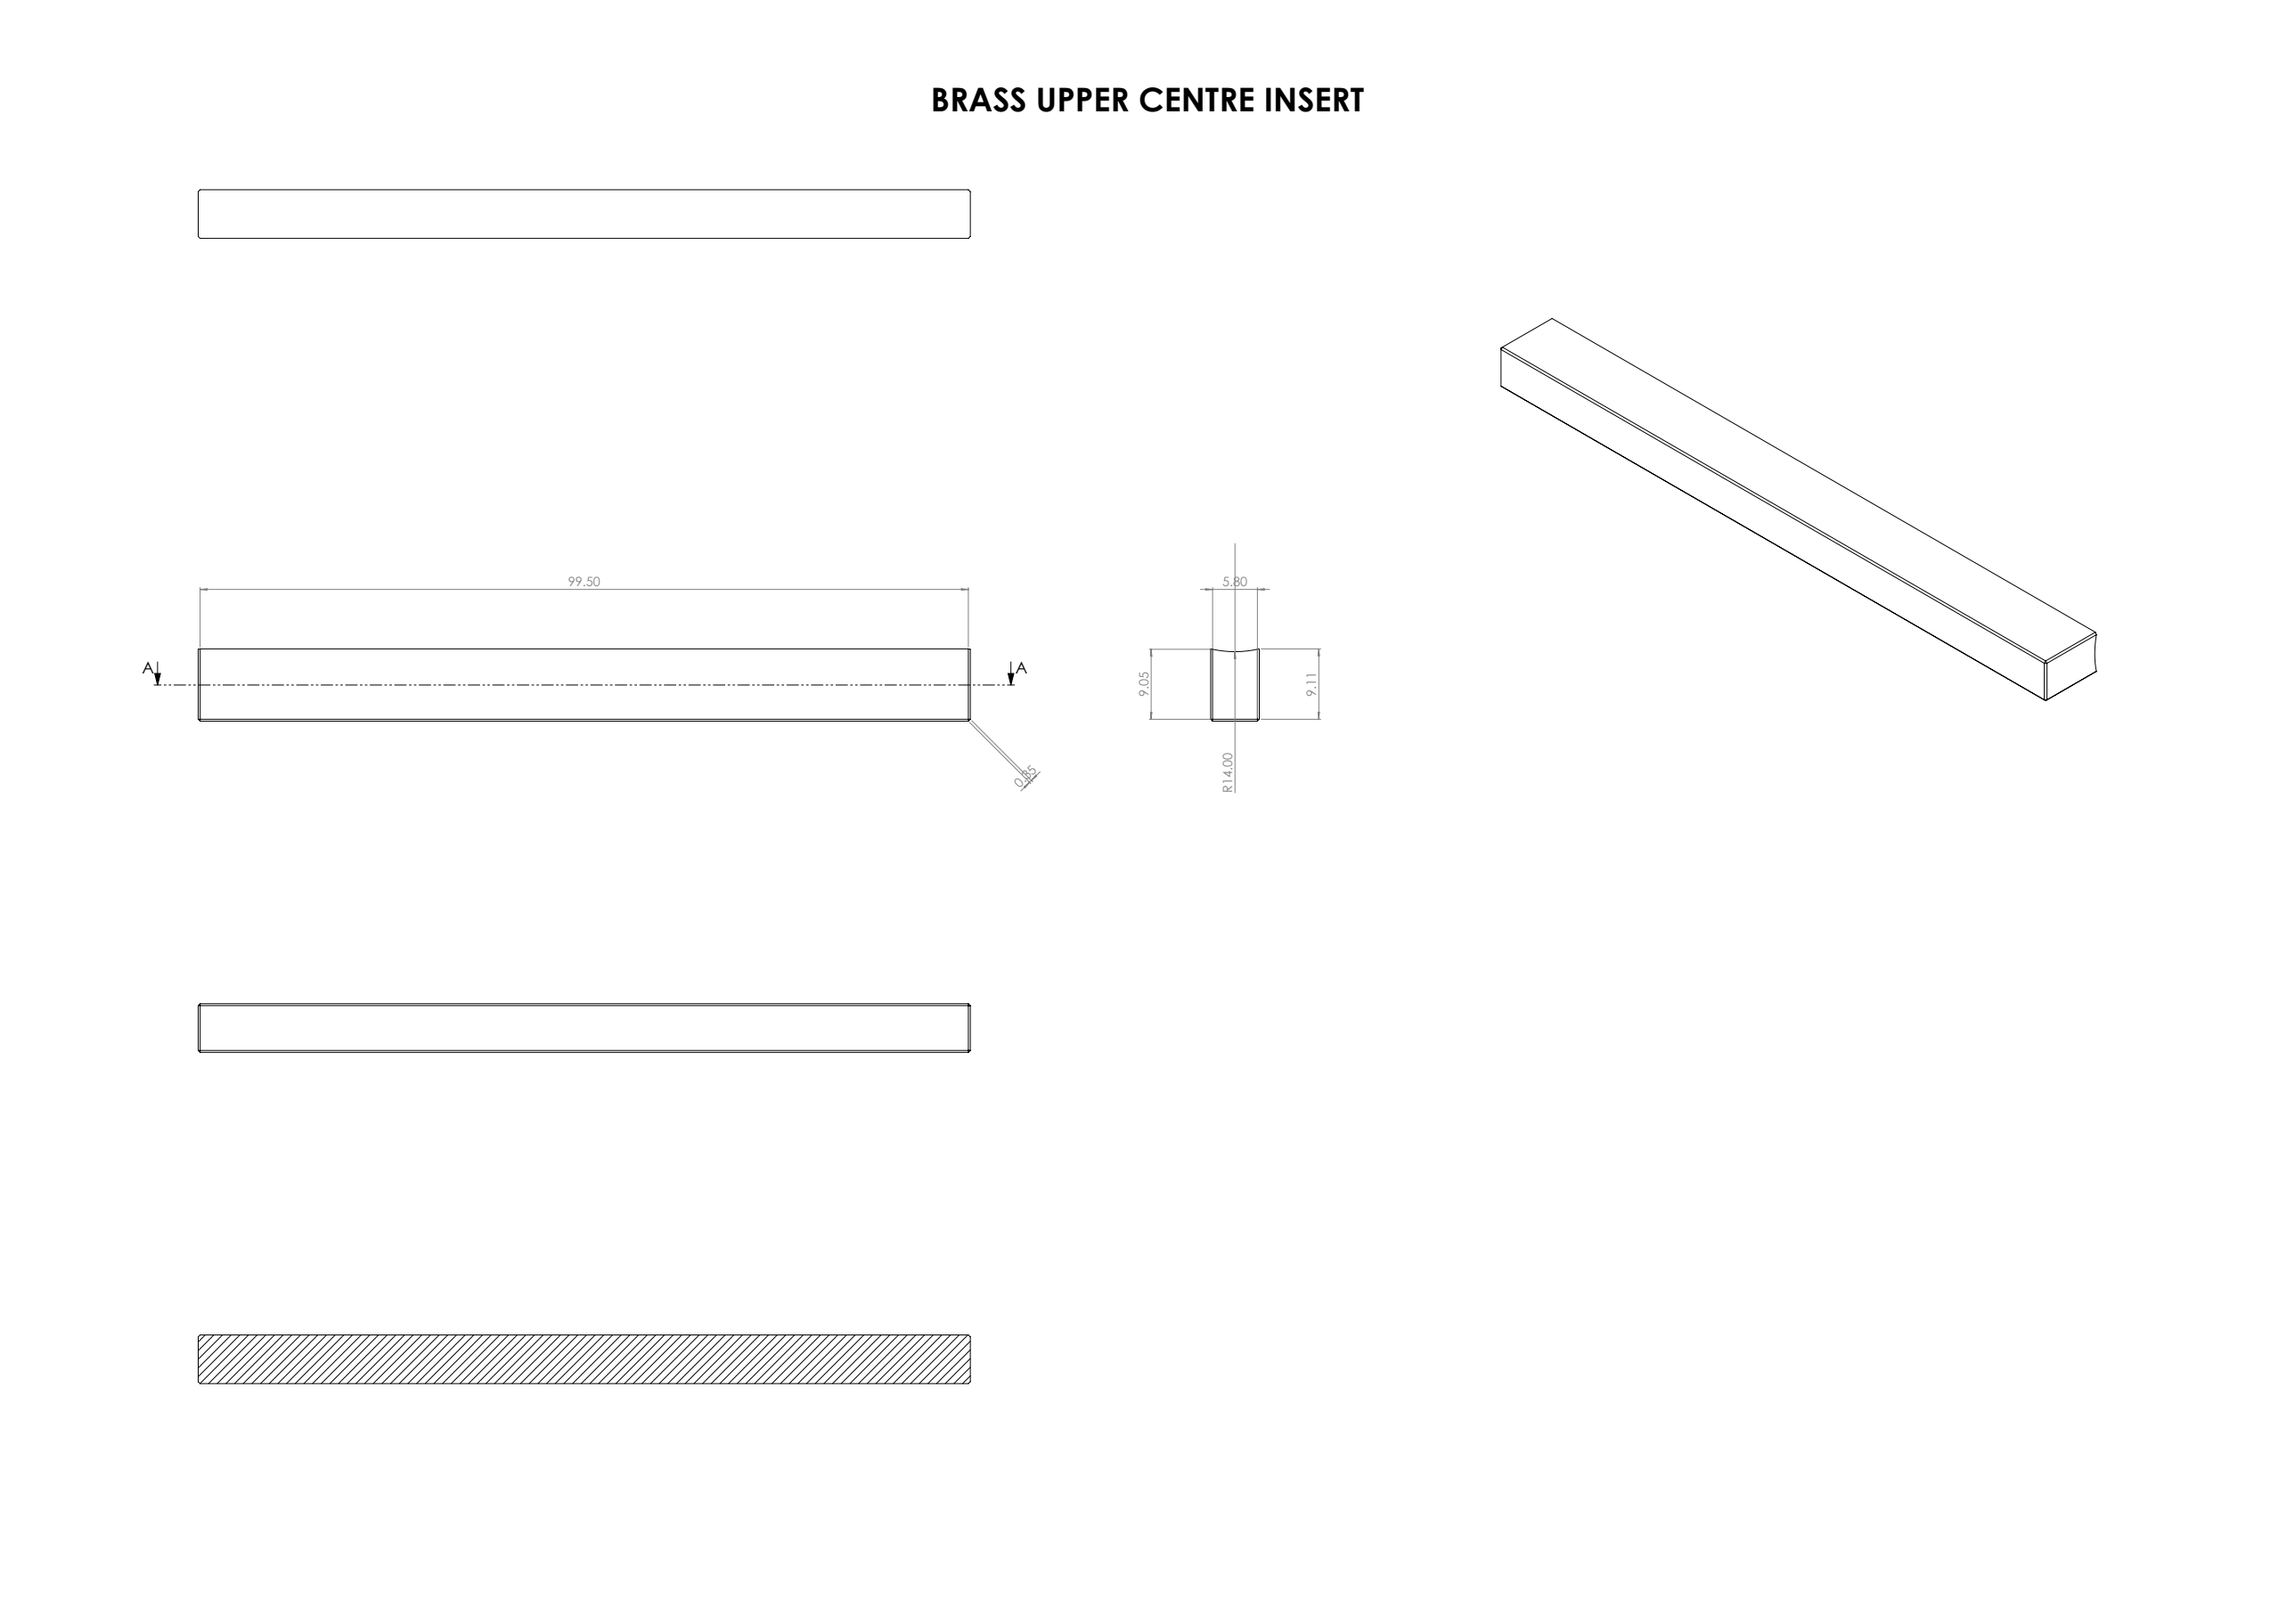
ISO-10303-21;
HEADER;
/* Generated by software containing ST-Developer
 * from STEP Tools, Inc. (www.steptools.com) 
 */

FILE_DESCRIPTION(
/* description */ (''),
/* implementation_level */ '2;1');

FILE_NAME(
/* name */ '13_Brass_Upper_Centre_Insert.step',
/* time_stamp */ '2026-10-21T01:59:45-07:00',
/* author */ (''),
/* organization */ (''),
/* preprocessor_version */ 'ST-DEVELOPER v20.2',
/* originating_system */ 'Autodesk Translation Framework v15.15.0.0',
/* authorisation */ '');

FILE_SCHEMA (('AUTOMOTIVE_DESIGN { 1 0 10303 214 3 1 1 }'));
ENDSEC;

DATA;
#10=MECHANICAL_DESIGN_GEOMETRIC_PRESENTATION_REPRESENTATION('',(#464),#18281);
#438=SHAPE_REPRESENTATION_RELATIONSHIP('SRR','None',#18340,#451);
#451=ADVANCED_BREP_SHAPE_REPRESENTATION('',(#482),#18269);
#464=STYLED_ITEM('',(#18467),#482);
#482=MANIFOLD_SOLID_BREP('Body1',#9086);
#498=CYLINDRICAL_SURFACE('',#9298,14.);
#637=CIRCLE('',#9296,14.);
#638=CIRCLE('',#9299,14.);
#826=ELLIPSE('',#9281,19.7989898732233,14.);
#827=ELLIPSE('',#9286,19.7989898732233,14.);
#828=ELLIPSE('',#9291,19.7989898732235,14.);
#829=ELLIPSE('',#9293,19.7989898732235,14.);
#863=FACE_OUTER_BOUND('',#1391,.T.);
#864=FACE_OUTER_BOUND('',#1392,.T.);
#865=FACE_OUTER_BOUND('',#1393,.T.);
#866=FACE_OUTER_BOUND('',#1394,.T.);
#867=FACE_OUTER_BOUND('',#1395,.T.);
#868=FACE_OUTER_BOUND('',#1396,.T.);
#869=FACE_OUTER_BOUND('',#1397,.T.);
#870=FACE_OUTER_BOUND('',#1398,.T.);
#871=FACE_OUTER_BOUND('',#1399,.T.);
#872=FACE_OUTER_BOUND('',#1400,.T.);
#873=FACE_OUTER_BOUND('',#1401,.T.);
#874=FACE_OUTER_BOUND('',#1402,.T.);
#875=FACE_OUTER_BOUND('',#1403,.T.);
#876=FACE_OUTER_BOUND('',#1404,.T.);
#877=FACE_OUTER_BOUND('',#1405,.T.);
#878=FACE_OUTER_BOUND('',#1406,.T.);
#879=FACE_OUTER_BOUND('',#1407,.T.);
#880=FACE_OUTER_BOUND('',#1408,.T.);
#1391=EDGE_LOOP('',(#5782,#5783,#5784));
#1392=EDGE_LOOP('',(#5785,#5786,#5787));
#1393=EDGE_LOOP('',(#5788,#5789,#5790,#5791));
#1394=EDGE_LOOP('',(#5792,#5793,#5794,#5795));
#1395=EDGE_LOOP('',(#5796,#5797,#5798));
#1396=EDGE_LOOP('',(#5799,#5800,#5801));
#1397=EDGE_LOOP('',(#5802,#5803,#5804,#5805));
#1398=EDGE_LOOP('',(#5806,#5807,#5808,#5809));
#1399=EDGE_LOOP('',(#5810,#5811,#5812,#5813));
#1400=EDGE_LOOP('',(#5814,#5815,#5816,#5817));
#1401=EDGE_LOOP('',(#5818,#5819,#5820,#5821));
#1402=EDGE_LOOP('',(#5822,#5823,#5824,#5825));
#1403=EDGE_LOOP('',(#5826,#5827,#5828,#5829));
#1404=EDGE_LOOP('',(#5830,#5831,#5832,#5833));
#1405=EDGE_LOOP('',(#5834,#5835,#5836,#5837));
#1406=EDGE_LOOP('',(#5838,#5839,#5840,#5841,#5842,#5843,#5844,#5845));
#1407=EDGE_LOOP('',(#5846,#5847,#5848,#5849));
#1408=EDGE_LOOP('',(#5850,#5851,#5852,#5853));
#1969=LINE('',#12369,#2814);
#1970=LINE('',#12371,#2815);
#1971=LINE('',#12372,#2816);
#1972=LINE('',#12376,#2817);
#1973=LINE('',#12378,#2818);
#1974=LINE('',#12379,#2819);
#1975=LINE('',#12384,#2820);
#1976=LINE('',#12385,#2821);
#1977=LINE('',#12387,#2822);
#1978=LINE('',#12388,#2823);
#1979=LINE('',#12392,#2824);
#1980=LINE('',#12394,#2825);
#1981=LINE('',#12395,#2826);
#1982=LINE('',#12399,#2827);
#1983=LINE('',#12401,#2828);
#1984=LINE('',#12402,#2829);
#1985=LINE('',#12407,#2830);
#1986=LINE('',#12408,#2831);
#1987=LINE('',#12410,#2832);
#1988=LINE('',#12411,#2833);
#1989=LINE('',#12413,#2834);
#1990=LINE('',#12414,#2835);
#1991=LINE('',#12416,#2836);
#1992=LINE('',#12417,#2837);
#1993=LINE('',#12422,#2838);
#1994=LINE('',#12423,#2839);
#1995=LINE('',#12428,#2840);
#1996=LINE('',#12429,#2841);
#1997=LINE('',#12431,#2842);
#1998=LINE('',#12436,#2843);
#2814=VECTOR('',#10077,10.);
#2815=VECTOR('',#10078,10.);
#2816=VECTOR('',#10079,10.);
#2817=VECTOR('',#10082,10.);
#2818=VECTOR('',#10083,10.);
#2819=VECTOR('',#10084,10.);
#2820=VECTOR('',#10089,10.);
#2821=VECTOR('',#10090,10.);
#2822=VECTOR('',#10093,10.);
#2823=VECTOR('',#10094,10.);
#2824=VECTOR('',#10097,10.);
#2825=VECTOR('',#10098,10.);
#2826=VECTOR('',#10099,10.);
#2827=VECTOR('',#10102,10.);
#2828=VECTOR('',#10103,10.);
#2829=VECTOR('',#10104,10.);
#2830=VECTOR('',#10109,10.);
#2831=VECTOR('',#10110,10.);
#2832=VECTOR('',#10113,10.);
#2833=VECTOR('',#10114,10.);
#2834=VECTOR('',#10117,10.);
#2835=VECTOR('',#10118,10.);
#2836=VECTOR('',#10121,10.);
#2837=VECTOR('',#10122,10.);
#2838=VECTOR('',#10127,10.);
#2839=VECTOR('',#10128,10.);
#2840=VECTOR('',#10133,10.);
#2841=VECTOR('',#10134,10.);
#2842=VECTOR('',#10137,10.);
#2843=VECTOR('',#10146,10.);
#3652=VERTEX_POINT('',#12367);
#3653=VERTEX_POINT('',#12368);
#3654=VERTEX_POINT('',#12370);
#3655=VERTEX_POINT('',#12374);
#3656=VERTEX_POINT('',#12375);
#3657=VERTEX_POINT('',#12377);
#3658=VERTEX_POINT('',#12381);
#3659=VERTEX_POINT('',#12382);
#3660=VERTEX_POINT('',#12390);
#3661=VERTEX_POINT('',#12391);
#3662=VERTEX_POINT('',#12393);
#3663=VERTEX_POINT('',#12397);
#3664=VERTEX_POINT('',#12398);
#3665=VERTEX_POINT('',#12400);
#3666=VERTEX_POINT('',#12404);
#3667=VERTEX_POINT('',#12405);
#3668=VERTEX_POINT('',#12419);
#3669=VERTEX_POINT('',#12420);
#3670=VERTEX_POINT('',#12425);
#3671=VERTEX_POINT('',#12426);
#4463=EDGE_CURVE('',#3652,#3653,#1969,.T.);
#4464=EDGE_CURVE('',#3654,#3652,#1970,.T.);
#4465=EDGE_CURVE('',#3653,#3654,#1971,.T.);
#4466=EDGE_CURVE('',#3655,#3656,#1972,.T.);
#4467=EDGE_CURVE('',#3657,#3655,#1973,.T.);
#4468=EDGE_CURVE('',#3656,#3657,#1974,.T.);
#4469=EDGE_CURVE('',#3658,#3659,#826,.T.);
#4470=EDGE_CURVE('',#3659,#3657,#1975,.T.);
#4471=EDGE_CURVE('',#3655,#3658,#1976,.T.);
#4472=EDGE_CURVE('',#3652,#3656,#1977,.T.);
#4473=EDGE_CURVE('',#3657,#3654,#1978,.T.);
#4474=EDGE_CURVE('',#3660,#3661,#1979,.T.);
#4475=EDGE_CURVE('',#3662,#3660,#1980,.T.);
#4476=EDGE_CURVE('',#3661,#3662,#1981,.T.);
#4477=EDGE_CURVE('',#3663,#3664,#1982,.T.);
#4478=EDGE_CURVE('',#3665,#3663,#1983,.T.);
#4479=EDGE_CURVE('',#3664,#3665,#1984,.T.);
#4480=EDGE_CURVE('',#3666,#3667,#827,.T.);
#4481=EDGE_CURVE('',#3667,#3665,#1985,.T.);
#4482=EDGE_CURVE('',#3663,#3666,#1986,.T.);
#4483=EDGE_CURVE('',#3656,#3664,#1987,.T.);
#4484=EDGE_CURVE('',#3665,#3655,#1988,.T.);
#4485=EDGE_CURVE('',#3660,#3663,#1989,.T.);
#4486=EDGE_CURVE('',#3664,#3662,#1990,.T.);
#4487=EDGE_CURVE('',#3653,#3661,#1991,.T.);
#4488=EDGE_CURVE('',#3662,#3652,#1992,.T.);
#4489=EDGE_CURVE('',#3668,#3669,#828,.T.);
#4490=EDGE_CURVE('',#3669,#3660,#1993,.T.);
#4491=EDGE_CURVE('',#3661,#3668,#1994,.T.);
#4492=EDGE_CURVE('',#3670,#3671,#829,.T.);
#4493=EDGE_CURVE('',#3671,#3653,#1995,.T.);
#4494=EDGE_CURVE('',#3654,#3670,#1996,.T.);
#4495=EDGE_CURVE('',#3669,#3666,#1997,.T.);
#4496=EDGE_CURVE('',#3671,#3668,#637,.T.);
#4497=EDGE_CURVE('',#3659,#3670,#1998,.T.);
#4498=EDGE_CURVE('',#3667,#3658,#638,.T.);
#5782=ORIENTED_EDGE('',*,*,#4463,.F.);
#5783=ORIENTED_EDGE('',*,*,#4464,.F.);
#5784=ORIENTED_EDGE('',*,*,#4465,.F.);
#5785=ORIENTED_EDGE('',*,*,#4466,.F.);
#5786=ORIENTED_EDGE('',*,*,#4467,.F.);
#5787=ORIENTED_EDGE('',*,*,#4468,.F.);
#5788=ORIENTED_EDGE('',*,*,#4469,.T.);
#5789=ORIENTED_EDGE('',*,*,#4470,.T.);
#5790=ORIENTED_EDGE('',*,*,#4467,.T.);
#5791=ORIENTED_EDGE('',*,*,#4471,.T.);
#5792=ORIENTED_EDGE('',*,*,#4464,.T.);
#5793=ORIENTED_EDGE('',*,*,#4472,.T.);
#5794=ORIENTED_EDGE('',*,*,#4468,.T.);
#5795=ORIENTED_EDGE('',*,*,#4473,.T.);
#5796=ORIENTED_EDGE('',*,*,#4474,.F.);
#5797=ORIENTED_EDGE('',*,*,#4475,.F.);
#5798=ORIENTED_EDGE('',*,*,#4476,.F.);
#5799=ORIENTED_EDGE('',*,*,#4477,.F.);
#5800=ORIENTED_EDGE('',*,*,#4478,.F.);
#5801=ORIENTED_EDGE('',*,*,#4479,.F.);
#5802=ORIENTED_EDGE('',*,*,#4480,.T.);
#5803=ORIENTED_EDGE('',*,*,#4481,.T.);
#5804=ORIENTED_EDGE('',*,*,#4478,.T.);
#5805=ORIENTED_EDGE('',*,*,#4482,.T.);
#5806=ORIENTED_EDGE('',*,*,#4466,.T.);
#5807=ORIENTED_EDGE('',*,*,#4483,.T.);
#5808=ORIENTED_EDGE('',*,*,#4479,.T.);
#5809=ORIENTED_EDGE('',*,*,#4484,.T.);
#5810=ORIENTED_EDGE('',*,*,#4475,.T.);
#5811=ORIENTED_EDGE('',*,*,#4485,.T.);
#5812=ORIENTED_EDGE('',*,*,#4477,.T.);
#5813=ORIENTED_EDGE('',*,*,#4486,.T.);
#5814=ORIENTED_EDGE('',*,*,#4463,.T.);
#5815=ORIENTED_EDGE('',*,*,#4487,.T.);
#5816=ORIENTED_EDGE('',*,*,#4476,.T.);
#5817=ORIENTED_EDGE('',*,*,#4488,.T.);
#5818=ORIENTED_EDGE('',*,*,#4489,.T.);
#5819=ORIENTED_EDGE('',*,*,#4490,.T.);
#5820=ORIENTED_EDGE('',*,*,#4474,.T.);
#5821=ORIENTED_EDGE('',*,*,#4491,.T.);
#5822=ORIENTED_EDGE('',*,*,#4492,.T.);
#5823=ORIENTED_EDGE('',*,*,#4493,.T.);
#5824=ORIENTED_EDGE('',*,*,#4465,.T.);
#5825=ORIENTED_EDGE('',*,*,#4494,.T.);
#5826=ORIENTED_EDGE('',*,*,#4482,.F.);
#5827=ORIENTED_EDGE('',*,*,#4485,.F.);
#5828=ORIENTED_EDGE('',*,*,#4490,.F.);
#5829=ORIENTED_EDGE('',*,*,#4495,.T.);
#5830=ORIENTED_EDGE('',*,*,#4491,.F.);
#5831=ORIENTED_EDGE('',*,*,#4487,.F.);
#5832=ORIENTED_EDGE('',*,*,#4493,.F.);
#5833=ORIENTED_EDGE('',*,*,#4496,.T.);
#5834=ORIENTED_EDGE('',*,*,#4472,.F.);
#5835=ORIENTED_EDGE('',*,*,#4488,.F.);
#5836=ORIENTED_EDGE('',*,*,#4486,.F.);
#5837=ORIENTED_EDGE('',*,*,#4483,.F.);
#5838=ORIENTED_EDGE('',*,*,#4480,.F.);
#5839=ORIENTED_EDGE('',*,*,#4495,.F.);
#5840=ORIENTED_EDGE('',*,*,#4489,.F.);
#5841=ORIENTED_EDGE('',*,*,#4496,.F.);
#5842=ORIENTED_EDGE('',*,*,#4492,.F.);
#5843=ORIENTED_EDGE('',*,*,#4497,.F.);
#5844=ORIENTED_EDGE('',*,*,#4469,.F.);
#5845=ORIENTED_EDGE('',*,*,#4498,.F.);
#5846=ORIENTED_EDGE('',*,*,#4481,.F.);
#5847=ORIENTED_EDGE('',*,*,#4498,.T.);
#5848=ORIENTED_EDGE('',*,*,#4471,.F.);
#5849=ORIENTED_EDGE('',*,*,#4484,.F.);
#5850=ORIENTED_EDGE('',*,*,#4470,.F.);
#5851=ORIENTED_EDGE('',*,*,#4497,.T.);
#5852=ORIENTED_EDGE('',*,*,#4494,.F.);
#5853=ORIENTED_EDGE('',*,*,#4473,.F.);
#8257=PLANE('',#9278);
#8258=PLANE('',#9279);
#8259=PLANE('',#9280);
#8260=PLANE('',#9282);
#8261=PLANE('',#9283);
#8262=PLANE('',#9284);
#8263=PLANE('',#9285);
#8264=PLANE('',#9287);
#8265=PLANE('',#9288);
#8266=PLANE('',#9289);
#8267=PLANE('',#9290);
#8268=PLANE('',#9292);
#8269=PLANE('',#9294);
#8270=PLANE('',#9295);
#8271=PLANE('',#9297);
#8272=PLANE('',#9300);
#8273=PLANE('',#9301);
#8584=ADVANCED_FACE('',(#863),#8257,.T.);
#8585=ADVANCED_FACE('',(#864),#8258,.T.);
#8586=ADVANCED_FACE('',(#865),#8259,.T.);
#8587=ADVANCED_FACE('',(#866),#8260,.T.);
#8588=ADVANCED_FACE('',(#867),#8261,.T.);
#8589=ADVANCED_FACE('',(#868),#8262,.T.);
#8590=ADVANCED_FACE('',(#869),#8263,.T.);
#8591=ADVANCED_FACE('',(#870),#8264,.T.);
#8592=ADVANCED_FACE('',(#871),#8265,.T.);
#8593=ADVANCED_FACE('',(#872),#8266,.T.);
#8594=ADVANCED_FACE('',(#873),#8267,.T.);
#8595=ADVANCED_FACE('',(#874),#8268,.T.);
#8596=ADVANCED_FACE('',(#875),#8269,.T.);
#8597=ADVANCED_FACE('',(#876),#8270,.T.);
#8598=ADVANCED_FACE('',(#877),#8271,.T.);
#8599=ADVANCED_FACE('',(#878),#498,.F.);
#8600=ADVANCED_FACE('',(#879),#8272,.F.);
#8601=ADVANCED_FACE('',(#880),#8273,.T.);
#9086=CLOSED_SHELL('',(#8584,#8585,#8586,#8587,#8588,#8589,#8590,#8591,
#8592,#8593,#8594,#8595,#8596,#8597,#8598,#8599,#8600,#8601));
#9277=AXIS2_PLACEMENT_3D('',#12365,#10073,#10074);
#9278=AXIS2_PLACEMENT_3D('',#12366,#10075,#10076);
#9279=AXIS2_PLACEMENT_3D('',#12373,#10080,#10081);
#9280=AXIS2_PLACEMENT_3D('',#12380,#10085,#10086);
#9281=AXIS2_PLACEMENT_3D('',#12383,#10087,#10088);
#9282=AXIS2_PLACEMENT_3D('',#12386,#10091,#10092);
#9283=AXIS2_PLACEMENT_3D('',#12389,#10095,#10096);
#9284=AXIS2_PLACEMENT_3D('',#12396,#10100,#10101);
#9285=AXIS2_PLACEMENT_3D('',#12403,#10105,#10106);
#9286=AXIS2_PLACEMENT_3D('',#12406,#10107,#10108);
#9287=AXIS2_PLACEMENT_3D('',#12409,#10111,#10112);
#9288=AXIS2_PLACEMENT_3D('',#12412,#10115,#10116);
#9289=AXIS2_PLACEMENT_3D('',#12415,#10119,#10120);
#9290=AXIS2_PLACEMENT_3D('',#12418,#10123,#10124);
#9291=AXIS2_PLACEMENT_3D('',#12421,#10125,#10126);
#9292=AXIS2_PLACEMENT_3D('',#12424,#10129,#10130);
#9293=AXIS2_PLACEMENT_3D('',#12427,#10131,#10132);
#9294=AXIS2_PLACEMENT_3D('',#12430,#10135,#10136);
#9295=AXIS2_PLACEMENT_3D('',#12432,#10138,#10139);
#9296=AXIS2_PLACEMENT_3D('',#12433,#10140,#10141);
#9297=AXIS2_PLACEMENT_3D('',#12434,#10142,#10143);
#9298=AXIS2_PLACEMENT_3D('',#12435,#10144,#10145);
#9299=AXIS2_PLACEMENT_3D('',#12437,#10147,#10148);
#9300=AXIS2_PLACEMENT_3D('',#12438,#10149,#10150);
#9301=AXIS2_PLACEMENT_3D('',#12439,#10151,#10152);
#10073=DIRECTION('axis',(0.,0.,1.));
#10074=DIRECTION('refdir',(1.,0.,0.));
#10075=DIRECTION('center_axis',(0.577350269189623,-0.577350269189631,0.577350269189623));
#10076=DIRECTION('ref_axis',(0.707106781186548,0.,-0.707106781186548));
#10077=DIRECTION('',(0.707106781186547,0.,-0.707106781186547));
#10078=DIRECTION('',(0.,0.707106781186543,0.707106781186552));
#10079=DIRECTION('',(-0.707106781186552,-0.707106781186543,0.));
#10080=DIRECTION('center_axis',(-0.577350269189642,-0.577350269189621,0.577350269189614));
#10081=DIRECTION('ref_axis',(0.70710678118653,0.,0.707106781186565));
#10082=DIRECTION('',(0.70710678118653,0.,0.707106781186565));
#10083=DIRECTION('',(-0.707106781186547,0.707106781186548,-2.51214793389404E-14));
#10084=DIRECTION('',(0.,-0.707106781186543,-0.707106781186552));
#10085=DIRECTION('center_axis',(-0.707106781186548,-0.707106781186547,0.));
#10086=DIRECTION('ref_axis',(0.,0.,1.));
#10087=DIRECTION('center_axis',(0.707106781186548,0.707106781186547,0.));
#10088=DIRECTION('ref_axis',(-0.707106781186547,0.707106781186548,0.));
#10089=DIRECTION('',(0.,0.,1.));
#10090=DIRECTION('',(0.,0.,-1.));
#10091=DIRECTION('center_axis',(0.,-0.707106781186552,0.707106781186543));
#10092=DIRECTION('ref_axis',(1.,0.,0.));
#10093=DIRECTION('',(-1.,0.,0.));
#10094=DIRECTION('',(1.,0.,0.));
#10095=DIRECTION('center_axis',(0.577350269189623,0.577350269189631,0.577350269189623));
#10096=DIRECTION('ref_axis',(0.707106781186548,0.,-0.707106781186548));
#10097=DIRECTION('',(0.707106781186552,-0.707106781186543,0.));
#10098=DIRECTION('',(0.,0.707106781186543,-0.707106781186552));
#10099=DIRECTION('',(-0.707106781186547,0.,0.707106781186547));
#10100=DIRECTION('center_axis',(-0.577350269189642,0.577350269189621,0.577350269189614));
#10101=DIRECTION('ref_axis',(0.70710678118653,0.,0.707106781186565));
#10102=DIRECTION('',(0.,-0.707106781186543,0.707106781186552));
#10103=DIRECTION('',(0.707106781186547,0.707106781186548,2.51214793389404E-14));
#10104=DIRECTION('',(-0.70710678118653,0.,-0.707106781186565));
#10105=DIRECTION('center_axis',(-0.707106781186548,0.707106781186547,0.));
#10106=DIRECTION('ref_axis',(0.,0.,1.));
#10107=DIRECTION('center_axis',(0.707106781186548,-0.707106781186547,0.));
#10108=DIRECTION('ref_axis',(0.707106781186547,0.707106781186548,0.));
#10109=DIRECTION('',(0.,0.,1.));
#10110=DIRECTION('',(0.,0.,-1.));
#10111=DIRECTION('center_axis',(-0.707106781186565,0.,0.70710678118653));
#10112=DIRECTION('ref_axis',(0.70710678118653,0.,0.707106781186565));
#10113=DIRECTION('',(0.,1.,0.));
#10114=DIRECTION('',(0.,-1.,0.));
#10115=DIRECTION('center_axis',(0.,0.707106781186552,0.707106781186543));
#10116=DIRECTION('ref_axis',(1.,0.,0.));
#10117=DIRECTION('',(-1.,0.,0.));
#10118=DIRECTION('',(1.,0.,0.));
#10119=DIRECTION('center_axis',(0.707106781186548,0.,0.707106781186548));
#10120=DIRECTION('ref_axis',(0.707106781186548,0.,-0.707106781186548));
#10121=DIRECTION('',(0.,1.,0.));
#10122=DIRECTION('',(0.,-1.,0.));
#10123=DIRECTION('center_axis',(0.707106781186543,0.707106781186552,0.));
#10124=DIRECTION('ref_axis',(0.,0.,-1.));
#10125=DIRECTION('center_axis',(-0.707106781186543,-0.707106781186552,0.));
#10126=DIRECTION('ref_axis',(-0.707106781186552,0.707106781186543,0.));
#10127=DIRECTION('',(0.,0.,1.));
#10128=DIRECTION('',(0.,0.,-1.));
#10129=DIRECTION('center_axis',(0.707106781186543,-0.707106781186552,0.));
#10130=DIRECTION('ref_axis',(0.,0.,-1.));
#10131=DIRECTION('center_axis',(-0.707106781186543,0.707106781186552,0.));
#10132=DIRECTION('ref_axis',(0.707106781186552,0.707106781186543,0.));
#10133=DIRECTION('',(0.,0.,1.));
#10134=DIRECTION('',(0.,0.,-1.));
#10135=DIRECTION('center_axis',(0.,1.,0.));
#10136=DIRECTION('ref_axis',(0.,0.,1.));
#10137=DIRECTION('',(-1.,0.,0.));
#10138=DIRECTION('center_axis',(1.,0.,0.));
#10139=DIRECTION('ref_axis',(0.,0.,-1.));
#10140=DIRECTION('center_axis',(-1.,0.,0.));
#10141=DIRECTION('ref_axis',(0.,0.,-1.));
#10142=DIRECTION('center_axis',(0.,0.,1.));
#10143=DIRECTION('ref_axis',(0.,-1.,0.));
#10144=DIRECTION('center_axis',(1.,0.,0.));
#10145=DIRECTION('ref_axis',(0.,1.22464679914735E-16,1.));
#10146=DIRECTION('',(1.,0.,0.));
#10147=DIRECTION('center_axis',(1.,0.,0.));
#10148=DIRECTION('ref_axis',(0.,0.,-1.));
#10149=DIRECTION('center_axis',(1.,0.,0.));
#10150=DIRECTION('ref_axis',(0.,0.,-1.));
#10151=DIRECTION('center_axis',(0.,-1.,0.));
#10152=DIRECTION('ref_axis',(0.,0.,-1.));
#12365=CARTESIAN_POINT('',(0.,0.,0.));
#12366=CARTESIAN_POINT('Origin',(99.75,-3.15,70.25));
#12367=CARTESIAN_POINT('',(99.75,-2.9,70.5));
#12368=CARTESIAN_POINT('',(100.,-2.9,70.25));
#12369=CARTESIAN_POINT('',(99.75,-2.9,70.5));
#12370=CARTESIAN_POINT('',(99.75,-3.15,70.25));
#12371=CARTESIAN_POINT('',(99.75,-3.15,70.25));
#12372=CARTESIAN_POINT('',(100.,-2.9,70.25));
#12373=CARTESIAN_POINT('Origin',(0.25,-3.15,70.25));
#12374=CARTESIAN_POINT('',(0.,-2.9,70.25));
#12375=CARTESIAN_POINT('',(0.25,-2.9,70.5));
#12376=CARTESIAN_POINT('',(0.,-2.9,70.25));
#12377=CARTESIAN_POINT('',(0.25,-3.15,70.25));
#12378=CARTESIAN_POINT('',(0.25,-3.15,70.25));
#12379=CARTESIAN_POINT('',(0.25,-2.9,70.5));
#12380=CARTESIAN_POINT('Origin',(0.125,-3.025,67.5));
#12381=CARTESIAN_POINT('',(0.,-2.9,61.1963498787086));
#12382=CARTESIAN_POINT('',(0.25,-3.15,61.1410226889336));
#12383=CARTESIAN_POINT('Origin',(-2.9,0.,47.5));
#12384=CARTESIAN_POINT('',(0.25,-3.15,67.5));
#12385=CARTESIAN_POINT('',(0.,-2.9,67.5));
#12386=CARTESIAN_POINT('Origin',(0.,-3.025,70.375));
#12387=CARTESIAN_POINT('',(0.,-2.9,70.5));
#12388=CARTESIAN_POINT('',(0.,-3.15,70.25));
#12389=CARTESIAN_POINT('Origin',(99.75,2.9,70.5));
#12390=CARTESIAN_POINT('',(99.75,3.15,70.25));
#12391=CARTESIAN_POINT('',(100.,2.9,70.25));
#12392=CARTESIAN_POINT('',(99.75,3.15,70.25));
#12393=CARTESIAN_POINT('',(99.75,2.9,70.5));
#12394=CARTESIAN_POINT('',(99.75,2.9,70.5));
#12395=CARTESIAN_POINT('',(100.,2.9,70.25));
#12396=CARTESIAN_POINT('Origin',(0.,2.9,70.25));
#12397=CARTESIAN_POINT('',(0.25,3.15,70.25));
#12398=CARTESIAN_POINT('',(0.25,2.9,70.5));
#12399=CARTESIAN_POINT('',(0.25,3.15,70.25));
#12400=CARTESIAN_POINT('',(0.,2.9,70.25));
#12401=CARTESIAN_POINT('',(0.,2.9,70.25));
#12402=CARTESIAN_POINT('',(0.25,2.9,70.5));
#12403=CARTESIAN_POINT('Origin',(0.125,3.025,61.5));
#12404=CARTESIAN_POINT('',(0.25,3.15,61.1410226889336));
#12405=CARTESIAN_POINT('',(0.,2.9,61.1963498787086));
#12406=CARTESIAN_POINT('Origin',(-2.9,0.,47.5));
#12407=CARTESIAN_POINT('',(0.,2.9,61.5));
#12408=CARTESIAN_POINT('',(0.25,3.15,61.5));
#12409=CARTESIAN_POINT('Origin',(0.125,1.575,70.375));
#12410=CARTESIAN_POINT('',(0.25,1.575,70.5));
#12411=CARTESIAN_POINT('',(0.,1.575,70.25));
#12412=CARTESIAN_POINT('Origin',(0.,3.025,70.375));
#12413=CARTESIAN_POINT('',(0.,3.15,70.25));
#12414=CARTESIAN_POINT('',(0.,2.9,70.5));
#12415=CARTESIAN_POINT('Origin',(99.875,1.575,70.375));
#12416=CARTESIAN_POINT('',(100.,1.575,70.25));
#12417=CARTESIAN_POINT('',(99.75,1.575,70.5));
#12418=CARTESIAN_POINT('Origin',(99.875,3.025,61.5));
#12419=CARTESIAN_POINT('',(100.,2.9,61.1963498787086));
#12420=CARTESIAN_POINT('',(99.75,3.15,61.1410226889336));
#12421=CARTESIAN_POINT('Origin',(102.9,0.,47.5));
#12422=CARTESIAN_POINT('',(99.75,3.15,61.5));
#12423=CARTESIAN_POINT('',(100.,2.9,61.5));
#12424=CARTESIAN_POINT('Origin',(99.875,-3.025,67.5));
#12425=CARTESIAN_POINT('',(99.75,-3.15,61.1410226889336));
#12426=CARTESIAN_POINT('',(100.,-2.9,61.1963498787086));
#12427=CARTESIAN_POINT('Origin',(102.9,0.,47.5));
#12428=CARTESIAN_POINT('',(100.,-2.9,67.5));
#12429=CARTESIAN_POINT('',(99.75,-3.15,67.5));
#12430=CARTESIAN_POINT('Origin',(0.,3.15,58.5));
#12431=CARTESIAN_POINT('',(0.,3.15,61.1410226889336));
#12432=CARTESIAN_POINT('Origin',(100.,0.,64.5));
#12433=CARTESIAN_POINT('Origin',(100.,0.,47.5));
#12434=CARTESIAN_POINT('Origin',(0.,3.15,70.5));
#12435=CARTESIAN_POINT('Origin',(0.,0.,47.5));
#12436=CARTESIAN_POINT('',(0.,-3.15,61.1410226889336));
#12437=CARTESIAN_POINT('Origin',(0.,0.,47.5));
#12438=CARTESIAN_POINT('Origin',(0.,0.,64.5));
#12439=CARTESIAN_POINT('Origin',(0.,-3.15,70.5));
#18254=UNCERTAINTY_MEASURE_WITH_UNIT(LENGTH_MEASURE(0.01),#18282,
'DISTANCE_ACCURACY_VALUE',
'Maximum model space distance between geometric entities at asserted c
onnectivities');
#18266=UNCERTAINTY_MEASURE_WITH_UNIT(LENGTH_MEASURE(0.01),#18282,
'DISTANCE_ACCURACY_VALUE',
'Maximum model space distance between geometric entities at asserted c
onnectivities');
#18269=(
GEOMETRIC_REPRESENTATION_CONTEXT(3)
GLOBAL_UNCERTAINTY_ASSIGNED_CONTEXT((#18254))
GLOBAL_UNIT_ASSIGNED_CONTEXT((#18282,#18284,#18285))
REPRESENTATION_CONTEXT('','3D')
);
#18281=(
GEOMETRIC_REPRESENTATION_CONTEXT(3)
GLOBAL_UNCERTAINTY_ASSIGNED_CONTEXT((#18266))
GLOBAL_UNIT_ASSIGNED_CONTEXT((#18282,#18284,#18285))
REPRESENTATION_CONTEXT('','3D')
);
#18282=(
LENGTH_UNIT()
NAMED_UNIT(*)
SI_UNIT(.MILLI.,.METRE.)
);
#18284=(
NAMED_UNIT(*)
PLANE_ANGLE_UNIT()
SI_UNIT($,.RADIAN.)
);
#18285=(
NAMED_UNIT(*)
SI_UNIT($,.STERADIAN.)
SOLID_ANGLE_UNIT()
);
#18288=SHAPE_DEFINITION_REPRESENTATION(#18302,#18340);
#18302=PRODUCT_DEFINITION_SHAPE('',$,#18355);
#18340=SHAPE_REPRESENTATION('',(#9277),#18269);
#18352=PRODUCT_DEFINITION_CONTEXT('part definition',#18396,'design');
#18355=PRODUCT_DEFINITION('2026-10-20-13-03-18-173',
'13_Brass_Upper_Centre_Insert',#18369,#18352);
#18369=PRODUCT_DEFINITION_FORMATION('',$,#18400);
#18396=APPLICATION_CONTEXT(
'Core Data for Automotive Mechanical Design Process');
#18397=PRODUCT_CONTEXT('part definition',#18396,'mechanical');
#18400=PRODUCT('2026-10-20-13-03-18-173','13_Brass_Upper_Centre_Insert',
$,(#18397));
#18461=COLOUR_RGB('Sky Blue',0.24,0.69,0.87);
#18462=FILL_AREA_STYLE_COLOUR('',#18461);
#18463=FILL_AREA_STYLE('',(#18462));
#18464=SURFACE_STYLE_FILL_AREA(#18463);
#18465=SURFACE_SIDE_STYLE('',(#18464));
#18466=SURFACE_STYLE_USAGE(.BOTH.,#18465);
#18467=PRESENTATION_STYLE_ASSIGNMENT((#18466));
ENDSEC;
END-ISO-10303-21;
